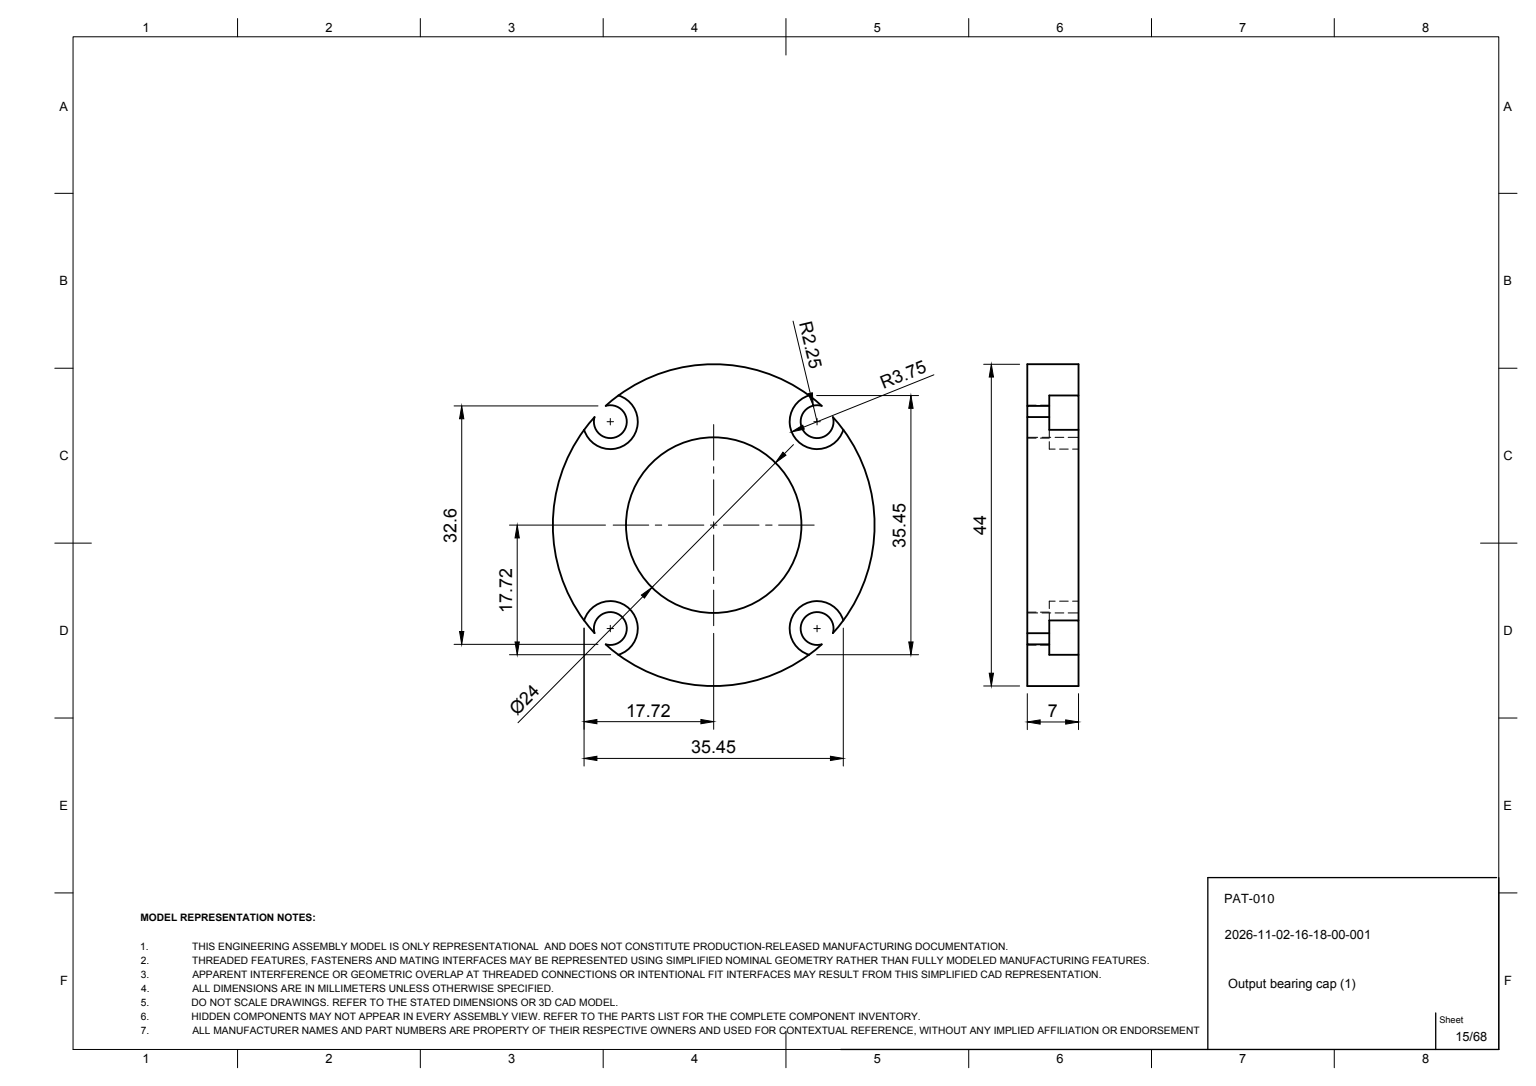
ISO-10303-21;
HEADER;
/* Generated by software containing ST-Developer
 * from STEP Tools, Inc. (www.steptools.com) 
 */

FILE_DESCRIPTION(
/* description */ ('Belt conveyor head drive unit'),
/* implementation_level */ '2;1');

FILE_NAME(
/* name */ 'Output bearing cap (1).step',
/* time_stamp */ '2026-10-28T03:26:19-07:00',
/* author */ (''),
/* organization */ (''),
/* preprocessor_version */ 'ST-DEVELOPER v20.2',
/* originating_system */ 'Autodesk Translation Framework v15.17.0.0',
/* authorisation */ '');

FILE_SCHEMA (('AUTOMOTIVE_DESIGN { 1 0 10303 214 3 1 1 }'));
ENDSEC;

DATA;
#10=MECHANICAL_DESIGN_GEOMETRIC_PRESENTATION_REPRESENTATION('',(#861),#27069);
#723=SHAPE_REPRESENTATION_RELATIONSHIP('SRR','None',#27367,#792);
#792=ADVANCED_BREP_SHAPE_REPRESENTATION('',(#946),#27009);
#861=STYLED_ITEM('',(#27797),#946);
#946=MANIFOLD_SOLID_BREP('Body1',#13726);
#1089=FACE_BOUND('',#2692,.T.);
#1090=FACE_BOUND('',#2694,.T.);
#1361=PLANE('',#14925);
#1362=PLANE('',#14929);
#1363=PLANE('',#14936);
#1364=PLANE('',#14943);
#1365=PLANE('',#14959);
#1366=PLANE('',#14964);
#1802=FACE_OUTER_BOUND('',#2679,.T.);
#1803=FACE_OUTER_BOUND('',#2680,.T.);
#1804=FACE_OUTER_BOUND('',#2681,.T.);
#1805=FACE_OUTER_BOUND('',#2682,.T.);
#1806=FACE_OUTER_BOUND('',#2683,.T.);
#1807=FACE_OUTER_BOUND('',#2684,.T.);
#1808=FACE_OUTER_BOUND('',#2685,.T.);
#1809=FACE_OUTER_BOUND('',#2686,.T.);
#1810=FACE_OUTER_BOUND('',#2687,.T.);
#1811=FACE_OUTER_BOUND('',#2688,.T.);
#1812=FACE_OUTER_BOUND('',#2689,.T.);
#1813=FACE_OUTER_BOUND('',#2690,.T.);
#1814=FACE_OUTER_BOUND('',#2691,.T.);
#1815=FACE_OUTER_BOUND('',#2693,.T.);
#1816=FACE_OUTER_BOUND('',#2695,.T.);
#1817=FACE_OUTER_BOUND('',#2696,.T.);
#1818=FACE_OUTER_BOUND('',#2697,.T.);
#1819=FACE_OUTER_BOUND('',#2698,.T.);
#1820=FACE_OUTER_BOUND('',#2699,.T.);
#2679=EDGE_LOOP('',(#9714,#9715,#9716,#9717));
#2680=EDGE_LOOP('',(#9718,#9719,#9720,#9721));
#2681=EDGE_LOOP('',(#9722,#9723,#9724,#9725));
#2682=EDGE_LOOP('',(#9726,#9727,#9728,#9729));
#2683=EDGE_LOOP('',(#9730,#9731,#9732,#9733));
#2684=EDGE_LOOP('',(#9734,#9735,#9736,#9737));
#2685=EDGE_LOOP('',(#9738,#9739,#9740,#9741));
#2686=EDGE_LOOP('',(#9742,#9743,#9744,#9745));
#2687=EDGE_LOOP('',(#9746,#9747,#9748,#9749));
#2688=EDGE_LOOP('',(#9750,#9751,#9752,#9753));
#2689=EDGE_LOOP('',(#9754,#9755,#9756,#9757));
#2690=EDGE_LOOP('',(#9758,#9759,#9760,#9761,#9762,#9763,#9764,#9765));
#2691=EDGE_LOOP('',(#9766,#9767,#9768,#9769,#9770,#9771,#9772,#9773));
#2692=EDGE_LOOP('',(#9774));
#2693=EDGE_LOOP('',(#9775,#9776,#9777,#9778,#9779,#9780,#9781,#9782));
#2694=EDGE_LOOP('',(#9783));
#2695=EDGE_LOOP('',(#9784,#9785,#9786,#9787,#9788,#9789,#9790,#9791));
#2696=EDGE_LOOP('',(#9792,#9793,#9794,#9795,#9796,#9797,#9798,#9799));
#2697=EDGE_LOOP('',(#9800,#9801,#9802,#9803));
#2698=EDGE_LOOP('',(#9804,#9805,#9806,#9807,#9808,#9809,#9810,#9811));
#2699=EDGE_LOOP('',(#9812,#9813,#9814,#9815));
#3702=LINE('',#21789,#4494);
#3703=LINE('',#21793,#4495);
#3704=LINE('',#21812,#4496);
#3705=LINE('',#21815,#4497);
#3706=LINE('',#21827,#4498);
#3707=LINE('',#21830,#4499);
#3708=LINE('',#21842,#4500);
#3709=LINE('',#21845,#4501);
#3710=LINE('',#21848,#4502);
#3711=LINE('',#21851,#4503);
#3712=LINE('',#21854,#4504);
#3713=LINE('',#21857,#4505);
#3714=LINE('',#21860,#4506);
#3715=LINE('',#21863,#4507);
#3716=LINE('',#21868,#4508);
#3717=LINE('',#21886,#4509);
#3718=LINE('',#21889,#4510);
#4494=VECTOR('',#17360,1.);
#4495=VECTOR('',#17363,1.);
#4496=VECTOR('',#17386,1.);
#4497=VECTOR('',#17389,1.);
#4498=VECTOR('',#17402,1.);
#4499=VECTOR('',#17405,1.);
#4500=VECTOR('',#17418,1.);
#4501=VECTOR('',#17421,1.);
#4502=VECTOR('',#17424,1.);
#4503=VECTOR('',#17427,1.);
#4504=VECTOR('',#17430,1.);
#4505=VECTOR('',#17433,1.);
#4506=VECTOR('',#17436,1.);
#4507=VECTOR('',#17439,1.);
#4508=VECTOR('',#17446,1.);
#4509=VECTOR('',#17475,1.);
#4510=VECTOR('',#17480,1.2);
#5256=CIRCLE('',#14923,0.375);
#5257=CIRCLE('',#14924,0.375);
#5258=CIRCLE('',#14926,2.2);
#5259=CIRCLE('',#14927,0.225);
#5260=CIRCLE('',#14928,2.2);
#5261=CIRCLE('',#14930,2.2);
#5262=CIRCLE('',#14931,0.375);
#5263=CIRCLE('',#14932,2.2);
#5264=CIRCLE('',#14933,0.225);
#5265=CIRCLE('',#14935,0.375);
#5266=CIRCLE('',#14937,2.2);
#5267=CIRCLE('',#14938,0.375);
#5268=CIRCLE('',#14939,2.2);
#5269=CIRCLE('',#14940,0.225);
#5270=CIRCLE('',#14942,0.375);
#5271=CIRCLE('',#14944,2.2);
#5272=CIRCLE('',#14945,0.375);
#5273=CIRCLE('',#14946,2.2);
#5274=CIRCLE('',#14947,0.225);
#5275=CIRCLE('',#14949,0.375);
#5276=CIRCLE('',#14951,0.225);
#5277=CIRCLE('',#14953,0.225);
#5278=CIRCLE('',#14955,0.225);
#5279=CIRCLE('',#14957,2.2);
#5280=CIRCLE('',#14958,2.2);
#5281=CIRCLE('',#14960,2.2);
#5282=CIRCLE('',#14961,2.2);
#5283=CIRCLE('',#14962,2.2);
#5284=CIRCLE('',#14963,1.2);
#5285=CIRCLE('',#14965,0.225);
#5286=CIRCLE('',#14966,2.2);
#5287=CIRCLE('',#14967,2.2);
#5288=CIRCLE('',#14968,2.2);
#5289=CIRCLE('',#14969,1.2);
#6205=VERTEX_POINT('',#21787);
#6206=VERTEX_POINT('',#21788);
#6207=VERTEX_POINT('',#21790);
#6208=VERTEX_POINT('',#21792);
#6209=VERTEX_POINT('',#21796);
#6210=VERTEX_POINT('',#21798);
#6211=VERTEX_POINT('',#21802);
#6212=VERTEX_POINT('',#21803);
#6213=VERTEX_POINT('',#21805);
#6214=VERTEX_POINT('',#21807);
#6215=VERTEX_POINT('',#21811);
#6216=VERTEX_POINT('',#21813);
#6217=VERTEX_POINT('',#21817);
#6218=VERTEX_POINT('',#21818);
#6219=VERTEX_POINT('',#21820);
#6220=VERTEX_POINT('',#21822);
#6221=VERTEX_POINT('',#21826);
#6222=VERTEX_POINT('',#21828);
#6223=VERTEX_POINT('',#21832);
#6224=VERTEX_POINT('',#21833);
#6225=VERTEX_POINT('',#21835);
#6226=VERTEX_POINT('',#21837);
#6227=VERTEX_POINT('',#21841);
#6228=VERTEX_POINT('',#21843);
#6229=VERTEX_POINT('',#21847);
#6230=VERTEX_POINT('',#21849);
#6231=VERTEX_POINT('',#21853);
#6232=VERTEX_POINT('',#21855);
#6233=VERTEX_POINT('',#21859);
#6234=VERTEX_POINT('',#21861);
#6235=VERTEX_POINT('',#21866);
#6236=VERTEX_POINT('',#21873);
#6237=VERTEX_POINT('',#21876);
#6238=VERTEX_POINT('',#21881);
#7549=EDGE_CURVE('',#6205,#6206,#3702,.T.);
#7550=EDGE_CURVE('',#6207,#6205,#5256,.T.);
#7551=EDGE_CURVE('',#6208,#6207,#3703,.T.);
#7552=EDGE_CURVE('',#6206,#6208,#5257,.T.);
#7553=EDGE_CURVE('',#6209,#6205,#5258,.T.);
#7554=EDGE_CURVE('',#6210,#6209,#5259,.T.);
#7555=EDGE_CURVE('',#6207,#6210,#5260,.T.);
#7556=EDGE_CURVE('',#6211,#6212,#5261,.T.);
#7557=EDGE_CURVE('',#6211,#6213,#5262,.T.);
#7558=EDGE_CURVE('',#6214,#6213,#5263,.T.);
#7559=EDGE_CURVE('',#6212,#6214,#5264,.T.);
#7560=EDGE_CURVE('',#6215,#6211,#3704,.T.);
#7561=EDGE_CURVE('',#6216,#6215,#5265,.T.);
#7562=EDGE_CURVE('',#6213,#6216,#3705,.T.);
#7563=EDGE_CURVE('',#6217,#6218,#5266,.T.);
#7564=EDGE_CURVE('',#6217,#6219,#5267,.T.);
#7565=EDGE_CURVE('',#6220,#6219,#5268,.T.);
#7566=EDGE_CURVE('',#6218,#6220,#5269,.T.);
#7567=EDGE_CURVE('',#6221,#6217,#3706,.T.);
#7568=EDGE_CURVE('',#6222,#6221,#5270,.T.);
#7569=EDGE_CURVE('',#6219,#6222,#3707,.T.);
#7570=EDGE_CURVE('',#6223,#6224,#5271,.T.);
#7571=EDGE_CURVE('',#6223,#6225,#5272,.T.);
#7572=EDGE_CURVE('',#6226,#6225,#5273,.T.);
#7573=EDGE_CURVE('',#6224,#6226,#5274,.T.);
#7574=EDGE_CURVE('',#6227,#6223,#3708,.T.);
#7575=EDGE_CURVE('',#6228,#6227,#5275,.T.);
#7576=EDGE_CURVE('',#6225,#6228,#3709,.T.);
#7577=EDGE_CURVE('',#6229,#6214,#3710,.T.);
#7578=EDGE_CURVE('',#6230,#6229,#5276,.T.);
#7579=EDGE_CURVE('',#6212,#6230,#3711,.T.);
#7580=EDGE_CURVE('',#6231,#6220,#3712,.T.);
#7581=EDGE_CURVE('',#6232,#6231,#5277,.T.);
#7582=EDGE_CURVE('',#6218,#6232,#3713,.T.);
#7583=EDGE_CURVE('',#6233,#6226,#3714,.T.);
#7584=EDGE_CURVE('',#6234,#6233,#5278,.T.);
#7585=EDGE_CURVE('',#6224,#6234,#3715,.T.);
#7586=EDGE_CURVE('',#6227,#6206,#5279,.T.);
#7587=EDGE_CURVE('',#6234,#6235,#5280,.T.);
#7588=EDGE_CURVE('',#6235,#6209,#3716,.T.);
#7589=EDGE_CURVE('',#6208,#6216,#5281,.T.);
#7590=EDGE_CURVE('',#6215,#6222,#5282,.T.);
#7591=EDGE_CURVE('',#6221,#6228,#5283,.T.);
#7592=EDGE_CURVE('',#6236,#6236,#5284,.T.);
#7593=EDGE_CURVE('',#6237,#6235,#5285,.T.);
#7594=EDGE_CURVE('',#6232,#6233,#5286,.T.);
#7595=EDGE_CURVE('',#6230,#6231,#5287,.T.);
#7596=EDGE_CURVE('',#6237,#6229,#5288,.T.);
#7597=EDGE_CURVE('',#6238,#6238,#5289,.T.);
#7598=EDGE_CURVE('',#6210,#6237,#3717,.T.);
#7599=EDGE_CURVE('',#6236,#6238,#3718,.T.);
#9714=ORIENTED_EDGE('',*,*,#7549,.F.);
#9715=ORIENTED_EDGE('',*,*,#7550,.F.);
#9716=ORIENTED_EDGE('',*,*,#7551,.F.);
#9717=ORIENTED_EDGE('',*,*,#7552,.F.);
#9718=ORIENTED_EDGE('',*,*,#7553,.F.);
#9719=ORIENTED_EDGE('',*,*,#7554,.F.);
#9720=ORIENTED_EDGE('',*,*,#7555,.F.);
#9721=ORIENTED_EDGE('',*,*,#7550,.T.);
#9722=ORIENTED_EDGE('',*,*,#7556,.F.);
#9723=ORIENTED_EDGE('',*,*,#7557,.T.);
#9724=ORIENTED_EDGE('',*,*,#7558,.F.);
#9725=ORIENTED_EDGE('',*,*,#7559,.F.);
#9726=ORIENTED_EDGE('',*,*,#7560,.F.);
#9727=ORIENTED_EDGE('',*,*,#7561,.F.);
#9728=ORIENTED_EDGE('',*,*,#7562,.F.);
#9729=ORIENTED_EDGE('',*,*,#7557,.F.);
#9730=ORIENTED_EDGE('',*,*,#7563,.F.);
#9731=ORIENTED_EDGE('',*,*,#7564,.T.);
#9732=ORIENTED_EDGE('',*,*,#7565,.F.);
#9733=ORIENTED_EDGE('',*,*,#7566,.F.);
#9734=ORIENTED_EDGE('',*,*,#7567,.F.);
#9735=ORIENTED_EDGE('',*,*,#7568,.F.);
#9736=ORIENTED_EDGE('',*,*,#7569,.F.);
#9737=ORIENTED_EDGE('',*,*,#7564,.F.);
#9738=ORIENTED_EDGE('',*,*,#7570,.F.);
#9739=ORIENTED_EDGE('',*,*,#7571,.T.);
#9740=ORIENTED_EDGE('',*,*,#7572,.F.);
#9741=ORIENTED_EDGE('',*,*,#7573,.F.);
#9742=ORIENTED_EDGE('',*,*,#7574,.F.);
#9743=ORIENTED_EDGE('',*,*,#7575,.F.);
#9744=ORIENTED_EDGE('',*,*,#7576,.F.);
#9745=ORIENTED_EDGE('',*,*,#7571,.F.);
#9746=ORIENTED_EDGE('',*,*,#7559,.T.);
#9747=ORIENTED_EDGE('',*,*,#7577,.F.);
#9748=ORIENTED_EDGE('',*,*,#7578,.F.);
#9749=ORIENTED_EDGE('',*,*,#7579,.F.);
#9750=ORIENTED_EDGE('',*,*,#7566,.T.);
#9751=ORIENTED_EDGE('',*,*,#7580,.F.);
#9752=ORIENTED_EDGE('',*,*,#7581,.F.);
#9753=ORIENTED_EDGE('',*,*,#7582,.F.);
#9754=ORIENTED_EDGE('',*,*,#7573,.T.);
#9755=ORIENTED_EDGE('',*,*,#7583,.F.);
#9756=ORIENTED_EDGE('',*,*,#7584,.F.);
#9757=ORIENTED_EDGE('',*,*,#7585,.F.);
#9758=ORIENTED_EDGE('',*,*,#7553,.T.);
#9759=ORIENTED_EDGE('',*,*,#7549,.T.);
#9760=ORIENTED_EDGE('',*,*,#7586,.F.);
#9761=ORIENTED_EDGE('',*,*,#7574,.T.);
#9762=ORIENTED_EDGE('',*,*,#7570,.T.);
#9763=ORIENTED_EDGE('',*,*,#7585,.T.);
#9764=ORIENTED_EDGE('',*,*,#7587,.T.);
#9765=ORIENTED_EDGE('',*,*,#7588,.T.);
#9766=ORIENTED_EDGE('',*,*,#7552,.T.);
#9767=ORIENTED_EDGE('',*,*,#7589,.T.);
#9768=ORIENTED_EDGE('',*,*,#7561,.T.);
#9769=ORIENTED_EDGE('',*,*,#7590,.T.);
#9770=ORIENTED_EDGE('',*,*,#7568,.T.);
#9771=ORIENTED_EDGE('',*,*,#7591,.T.);
#9772=ORIENTED_EDGE('',*,*,#7575,.T.);
#9773=ORIENTED_EDGE('',*,*,#7586,.T.);
#9774=ORIENTED_EDGE('',*,*,#7592,.T.);
#9775=ORIENTED_EDGE('',*,*,#7593,.T.);
#9776=ORIENTED_EDGE('',*,*,#7587,.F.);
#9777=ORIENTED_EDGE('',*,*,#7584,.T.);
#9778=ORIENTED_EDGE('',*,*,#7594,.F.);
#9779=ORIENTED_EDGE('',*,*,#7581,.T.);
#9780=ORIENTED_EDGE('',*,*,#7595,.F.);
#9781=ORIENTED_EDGE('',*,*,#7578,.T.);
#9782=ORIENTED_EDGE('',*,*,#7596,.F.);
#9783=ORIENTED_EDGE('',*,*,#7597,.F.);
#9784=ORIENTED_EDGE('',*,*,#7563,.T.);
#9785=ORIENTED_EDGE('',*,*,#7582,.T.);
#9786=ORIENTED_EDGE('',*,*,#7594,.T.);
#9787=ORIENTED_EDGE('',*,*,#7583,.T.);
#9788=ORIENTED_EDGE('',*,*,#7572,.T.);
#9789=ORIENTED_EDGE('',*,*,#7576,.T.);
#9790=ORIENTED_EDGE('',*,*,#7591,.F.);
#9791=ORIENTED_EDGE('',*,*,#7567,.T.);
#9792=ORIENTED_EDGE('',*,*,#7556,.T.);
#9793=ORIENTED_EDGE('',*,*,#7579,.T.);
#9794=ORIENTED_EDGE('',*,*,#7595,.T.);
#9795=ORIENTED_EDGE('',*,*,#7580,.T.);
#9796=ORIENTED_EDGE('',*,*,#7565,.T.);
#9797=ORIENTED_EDGE('',*,*,#7569,.T.);
#9798=ORIENTED_EDGE('',*,*,#7590,.F.);
#9799=ORIENTED_EDGE('',*,*,#7560,.T.);
#9800=ORIENTED_EDGE('',*,*,#7554,.T.);
#9801=ORIENTED_EDGE('',*,*,#7588,.F.);
#9802=ORIENTED_EDGE('',*,*,#7593,.F.);
#9803=ORIENTED_EDGE('',*,*,#7598,.F.);
#9804=ORIENTED_EDGE('',*,*,#7555,.T.);
#9805=ORIENTED_EDGE('',*,*,#7598,.T.);
#9806=ORIENTED_EDGE('',*,*,#7596,.T.);
#9807=ORIENTED_EDGE('',*,*,#7577,.T.);
#9808=ORIENTED_EDGE('',*,*,#7558,.T.);
#9809=ORIENTED_EDGE('',*,*,#7562,.T.);
#9810=ORIENTED_EDGE('',*,*,#7589,.F.);
#9811=ORIENTED_EDGE('',*,*,#7551,.T.);
#9812=ORIENTED_EDGE('',*,*,#7592,.F.);
#9813=ORIENTED_EDGE('',*,*,#7599,.T.);
#9814=ORIENTED_EDGE('',*,*,#7597,.T.);
#9815=ORIENTED_EDGE('',*,*,#7599,.F.);
#12617=CYLINDRICAL_SURFACE('',#14922,0.375);
#12618=CYLINDRICAL_SURFACE('',#14934,0.375);
#12619=CYLINDRICAL_SURFACE('',#14941,0.375);
#12620=CYLINDRICAL_SURFACE('',#14948,0.375);
#12621=CYLINDRICAL_SURFACE('',#14950,0.225);
#12622=CYLINDRICAL_SURFACE('',#14952,0.225);
#12623=CYLINDRICAL_SURFACE('',#14954,0.225);
#12624=CYLINDRICAL_SURFACE('',#14956,2.2);
#12625=CYLINDRICAL_SURFACE('',#14970,2.2);
#12626=CYLINDRICAL_SURFACE('',#14971,2.2);
#12627=CYLINDRICAL_SURFACE('',#14972,0.225);
#12628=CYLINDRICAL_SURFACE('',#14973,2.2);
#12629=CYLINDRICAL_SURFACE('',#14974,1.2);
#13081=ADVANCED_FACE('',(#1802),#12617,.F.);
#13082=ADVANCED_FACE('',(#1803),#1361,.T.);
#13083=ADVANCED_FACE('',(#1804),#1362,.T.);
#13084=ADVANCED_FACE('',(#1805),#12618,.F.);
#13085=ADVANCED_FACE('',(#1806),#1363,.T.);
#13086=ADVANCED_FACE('',(#1807),#12619,.F.);
#13087=ADVANCED_FACE('',(#1808),#1364,.T.);
#13088=ADVANCED_FACE('',(#1809),#12620,.F.);
#13089=ADVANCED_FACE('',(#1810),#12621,.F.);
#13090=ADVANCED_FACE('',(#1811),#12622,.F.);
#13091=ADVANCED_FACE('',(#1812),#12623,.F.);
#13092=ADVANCED_FACE('',(#1813),#12624,.T.);
#13093=ADVANCED_FACE('',(#1814,#1089),#1365,.T.);
#13094=ADVANCED_FACE('',(#1815,#1090),#1366,.F.);
#13095=ADVANCED_FACE('',(#1816),#12625,.T.);
#13096=ADVANCED_FACE('',(#1817),#12626,.T.);
#13097=ADVANCED_FACE('',(#1818),#12627,.F.);
#13098=ADVANCED_FACE('',(#1819),#12628,.T.);
#13099=ADVANCED_FACE('',(#1820),#12629,.F.);
#13726=CLOSED_SHELL('',(#13081,#13082,#13083,#13084,#13085,#13086,#13087,
#13088,#13089,#13090,#13091,#13092,#13093,#13094,#13095,#13096,#13097,#13098,
#13099));
#14921=AXIS2_PLACEMENT_3D('',#21785,#17356,#17357);
#14922=AXIS2_PLACEMENT_3D('',#21786,#17358,#17359);
#14923=AXIS2_PLACEMENT_3D('',#21791,#17361,#17362);
#14924=AXIS2_PLACEMENT_3D('',#21794,#17364,#17365);
#14925=AXIS2_PLACEMENT_3D('',#21795,#17366,#17367);
#14926=AXIS2_PLACEMENT_3D('',#21797,#17368,#17369);
#14927=AXIS2_PLACEMENT_3D('',#21799,#17370,#17371);
#14928=AXIS2_PLACEMENT_3D('',#21800,#17372,#17373);
#14929=AXIS2_PLACEMENT_3D('',#21801,#17374,#17375);
#14930=AXIS2_PLACEMENT_3D('',#21804,#17376,#17377);
#14931=AXIS2_PLACEMENT_3D('',#21806,#17378,#17379);
#14932=AXIS2_PLACEMENT_3D('',#21808,#17380,#17381);
#14933=AXIS2_PLACEMENT_3D('',#21809,#17382,#17383);
#14934=AXIS2_PLACEMENT_3D('',#21810,#17384,#17385);
#14935=AXIS2_PLACEMENT_3D('',#21814,#17387,#17388);
#14936=AXIS2_PLACEMENT_3D('',#21816,#17390,#17391);
#14937=AXIS2_PLACEMENT_3D('',#21819,#17392,#17393);
#14938=AXIS2_PLACEMENT_3D('',#21821,#17394,#17395);
#14939=AXIS2_PLACEMENT_3D('',#21823,#17396,#17397);
#14940=AXIS2_PLACEMENT_3D('',#21824,#17398,#17399);
#14941=AXIS2_PLACEMENT_3D('',#21825,#17400,#17401);
#14942=AXIS2_PLACEMENT_3D('',#21829,#17403,#17404);
#14943=AXIS2_PLACEMENT_3D('',#21831,#17406,#17407);
#14944=AXIS2_PLACEMENT_3D('',#21834,#17408,#17409);
#14945=AXIS2_PLACEMENT_3D('',#21836,#17410,#17411);
#14946=AXIS2_PLACEMENT_3D('',#21838,#17412,#17413);
#14947=AXIS2_PLACEMENT_3D('',#21839,#17414,#17415);
#14948=AXIS2_PLACEMENT_3D('',#21840,#17416,#17417);
#14949=AXIS2_PLACEMENT_3D('',#21844,#17419,#17420);
#14950=AXIS2_PLACEMENT_3D('',#21846,#17422,#17423);
#14951=AXIS2_PLACEMENT_3D('',#21850,#17425,#17426);
#14952=AXIS2_PLACEMENT_3D('',#21852,#17428,#17429);
#14953=AXIS2_PLACEMENT_3D('',#21856,#17431,#17432);
#14954=AXIS2_PLACEMENT_3D('',#21858,#17434,#17435);
#14955=AXIS2_PLACEMENT_3D('',#21862,#17437,#17438);
#14956=AXIS2_PLACEMENT_3D('',#21864,#17440,#17441);
#14957=AXIS2_PLACEMENT_3D('',#21865,#17442,#17443);
#14958=AXIS2_PLACEMENT_3D('',#21867,#17444,#17445);
#14959=AXIS2_PLACEMENT_3D('',#21869,#17447,#17448);
#14960=AXIS2_PLACEMENT_3D('',#21870,#17449,#17450);
#14961=AXIS2_PLACEMENT_3D('',#21871,#17451,#17452);
#14962=AXIS2_PLACEMENT_3D('',#21872,#17453,#17454);
#14963=AXIS2_PLACEMENT_3D('',#21874,#17455,#17456);
#14964=AXIS2_PLACEMENT_3D('',#21875,#17457,#17458);
#14965=AXIS2_PLACEMENT_3D('',#21877,#17459,#17460);
#14966=AXIS2_PLACEMENT_3D('',#21878,#17461,#17462);
#14967=AXIS2_PLACEMENT_3D('',#21879,#17463,#17464);
#14968=AXIS2_PLACEMENT_3D('',#21880,#17465,#17466);
#14969=AXIS2_PLACEMENT_3D('',#21882,#17467,#17468);
#14970=AXIS2_PLACEMENT_3D('',#21883,#17469,#17470);
#14971=AXIS2_PLACEMENT_3D('',#21884,#17471,#17472);
#14972=AXIS2_PLACEMENT_3D('',#21885,#17473,#17474);
#14973=AXIS2_PLACEMENT_3D('',#21887,#17476,#17477);
#14974=AXIS2_PLACEMENT_3D('',#21888,#17478,#17479);
#17356=DIRECTION('axis',(0.,0.,1.));
#17357=DIRECTION('refdir',(1.,0.,0.));
#17358=DIRECTION('center_axis',(0.,1.,0.));
#17359=DIRECTION('ref_axis',(1.,0.,0.));
#17360=DIRECTION('',(0.,1.,0.));
#17361=DIRECTION('center_axis',(0.,1.,0.));
#17362=DIRECTION('ref_axis',(1.,0.,0.));
#17363=DIRECTION('',(0.,-1.,0.));
#17364=DIRECTION('center_axis',(0.,-1.,0.));
#17365=DIRECTION('ref_axis',(1.,0.,0.));
#17366=DIRECTION('center_axis',(0.,1.,0.));
#17367=DIRECTION('ref_axis',(1.,0.,0.));
#17368=DIRECTION('center_axis',(0.,-1.,0.));
#17369=DIRECTION('ref_axis',(1.,0.,0.));
#17370=DIRECTION('center_axis',(0.,1.,0.));
#17371=DIRECTION('ref_axis',(1.,0.,0.));
#17372=DIRECTION('center_axis',(0.,-1.,0.));
#17373=DIRECTION('ref_axis',(1.,0.,0.));
#17374=DIRECTION('center_axis',(0.,1.,0.));
#17375=DIRECTION('ref_axis',(1.,0.,0.));
#17376=DIRECTION('center_axis',(0.,-1.,0.));
#17377=DIRECTION('ref_axis',(1.,0.,0.));
#17378=DIRECTION('center_axis',(0.,1.,0.));
#17379=DIRECTION('ref_axis',(1.,0.,0.));
#17380=DIRECTION('center_axis',(0.,-1.,0.));
#17381=DIRECTION('ref_axis',(1.,0.,0.));
#17382=DIRECTION('center_axis',(0.,1.,0.));
#17383=DIRECTION('ref_axis',(1.,0.,0.));
#17384=DIRECTION('center_axis',(0.,1.,0.));
#17385=DIRECTION('ref_axis',(1.,0.,0.));
#17386=DIRECTION('',(0.,-1.,0.));
#17387=DIRECTION('center_axis',(0.,-1.,0.));
#17388=DIRECTION('ref_axis',(1.,0.,0.));
#17389=DIRECTION('',(0.,1.,0.));
#17390=DIRECTION('center_axis',(0.,1.,0.));
#17391=DIRECTION('ref_axis',(1.,0.,0.));
#17392=DIRECTION('center_axis',(0.,-1.,0.));
#17393=DIRECTION('ref_axis',(1.,0.,0.));
#17394=DIRECTION('center_axis',(0.,1.,0.));
#17395=DIRECTION('ref_axis',(1.,0.,0.));
#17396=DIRECTION('center_axis',(0.,-1.,0.));
#17397=DIRECTION('ref_axis',(1.,0.,0.));
#17398=DIRECTION('center_axis',(0.,1.,0.));
#17399=DIRECTION('ref_axis',(1.,0.,0.));
#17400=DIRECTION('center_axis',(0.,1.,0.));
#17401=DIRECTION('ref_axis',(-0.707106781186547,0.,-0.707106781186548));
#17402=DIRECTION('',(0.,-1.,0.));
#17403=DIRECTION('center_axis',(0.,-1.,0.));
#17404=DIRECTION('ref_axis',(1.,0.,0.));
#17405=DIRECTION('',(0.,1.,0.));
#17406=DIRECTION('center_axis',(0.,1.,0.));
#17407=DIRECTION('ref_axis',(1.,0.,0.));
#17408=DIRECTION('center_axis',(0.,-1.,0.));
#17409=DIRECTION('ref_axis',(1.,0.,0.));
#17410=DIRECTION('center_axis',(0.,1.,0.));
#17411=DIRECTION('ref_axis',(1.,0.,0.));
#17412=DIRECTION('center_axis',(0.,-1.,0.));
#17413=DIRECTION('ref_axis',(1.,0.,0.));
#17414=DIRECTION('center_axis',(0.,1.,0.));
#17415=DIRECTION('ref_axis',(1.,0.,0.));
#17416=DIRECTION('center_axis',(0.,1.,0.));
#17417=DIRECTION('ref_axis',(-0.707106781186548,0.,0.707106781186547));
#17418=DIRECTION('',(0.,-1.,0.));
#17419=DIRECTION('center_axis',(0.,-1.,0.));
#17420=DIRECTION('ref_axis',(1.,0.,0.));
#17421=DIRECTION('',(0.,1.,0.));
#17422=DIRECTION('center_axis',(0.,1.,0.));
#17423=DIRECTION('ref_axis',(0.707106781186545,0.,-0.70710678118655));
#17424=DIRECTION('',(0.,1.,0.));
#17425=DIRECTION('center_axis',(0.,1.,0.));
#17426=DIRECTION('ref_axis',(1.,0.,0.));
#17427=DIRECTION('',(0.,-1.,0.));
#17428=DIRECTION('center_axis',(0.,1.,0.));
#17429=DIRECTION('ref_axis',(-0.707106781186547,0.,-0.707106781186548));
#17430=DIRECTION('',(0.,1.,0.));
#17431=DIRECTION('center_axis',(0.,1.,0.));
#17432=DIRECTION('ref_axis',(1.,0.,0.));
#17433=DIRECTION('',(0.,-1.,0.));
#17434=DIRECTION('center_axis',(0.,1.,0.));
#17435=DIRECTION('ref_axis',(-0.707106781186544,0.,0.707106781186551));
#17436=DIRECTION('',(0.,1.,0.));
#17437=DIRECTION('center_axis',(0.,1.,0.));
#17438=DIRECTION('ref_axis',(1.,0.,0.));
#17439=DIRECTION('',(0.,-1.,0.));
#17440=DIRECTION('center_axis',(0.,1.,0.));
#17441=DIRECTION('ref_axis',(1.,0.,0.));
#17442=DIRECTION('center_axis',(0.,1.,0.));
#17443=DIRECTION('ref_axis',(1.,0.,0.));
#17444=DIRECTION('center_axis',(0.,1.,0.));
#17445=DIRECTION('ref_axis',(1.,0.,0.));
#17446=DIRECTION('',(0.,1.,0.));
#17447=DIRECTION('center_axis',(0.,1.,0.));
#17448=DIRECTION('ref_axis',(1.,0.,0.));
#17449=DIRECTION('center_axis',(0.,1.,0.));
#17450=DIRECTION('ref_axis',(1.,0.,0.));
#17451=DIRECTION('center_axis',(0.,1.,0.));
#17452=DIRECTION('ref_axis',(1.,0.,0.));
#17453=DIRECTION('center_axis',(0.,1.,0.));
#17454=DIRECTION('ref_axis',(1.,0.,0.));
#17455=DIRECTION('center_axis',(0.,-1.,0.));
#17456=DIRECTION('ref_axis',(1.,0.,0.));
#17457=DIRECTION('center_axis',(0.,1.,0.));
#17458=DIRECTION('ref_axis',(1.,0.,0.));
#17459=DIRECTION('center_axis',(0.,1.,0.));
#17460=DIRECTION('ref_axis',(1.,0.,0.));
#17461=DIRECTION('center_axis',(0.,1.,0.));
#17462=DIRECTION('ref_axis',(1.,0.,0.));
#17463=DIRECTION('center_axis',(0.,1.,0.));
#17464=DIRECTION('ref_axis',(1.,0.,0.));
#17465=DIRECTION('center_axis',(0.,1.,0.));
#17466=DIRECTION('ref_axis',(1.,0.,0.));
#17467=DIRECTION('center_axis',(0.,-1.,0.));
#17468=DIRECTION('ref_axis',(1.,0.,0.));
#17469=DIRECTION('center_axis',(0.,1.,0.));
#17470=DIRECTION('ref_axis',(1.,0.,0.));
#17471=DIRECTION('center_axis',(0.,1.,0.));
#17472=DIRECTION('ref_axis',(1.,0.,0.));
#17473=DIRECTION('center_axis',(0.,1.,0.));
#17474=DIRECTION('ref_axis',(0.707106781186544,0.,0.707106781186551));
#17475=DIRECTION('',(0.,-1.,0.));
#17476=DIRECTION('center_axis',(0.,1.,0.));
#17477=DIRECTION('ref_axis',(-1.,0.,-1.01064309961486E-15));
#17478=DIRECTION('center_axis',(0.,1.,0.));
#17479=DIRECTION('ref_axis',(1.,0.,0.));
#17480=DIRECTION('',(0.,-1.,0.));
#21785=CARTESIAN_POINT('',(0.,0.,0.));
#21786=CARTESIAN_POINT('Origin',(5.55669646780806,1.7,5.58578643762691));
#21787=CARTESIAN_POINT('',(5.66764231833408,1.7,5.22757418455471));
#21788=CARTESIAN_POINT('',(5.66764231833408,2.1,5.22757418455471));
#21789=CARTESIAN_POINT('',(5.66764231833408,1.7,5.22757418455471));
#21790=CARTESIAN_POINT('',(5.19848421473587,1.7,5.69673228815293));
#21791=CARTESIAN_POINT('Origin',(5.55669646780806,1.7,5.58578643762691));
#21792=CARTESIAN_POINT('',(5.19848421473587,2.1,5.69673228815293));
#21793=CARTESIAN_POINT('',(5.19848421473587,1.7,5.69673228815293));
#21794=CARTESIAN_POINT('Origin',(5.55669646780806,2.1,5.58578643762691));
#21795=CARTESIAN_POINT('Origin',(5.55669646780806,1.7,5.58578643762691));
#21796=CARTESIAN_POINT('',(5.49357471024299,1.7,5.36982198749241));
#21797=CARTESIAN_POINT('Origin',(6.97091003018116,1.7,7.));
#21798=CARTESIAN_POINT('',(5.34073201767356,1.7,5.52266468006184));
#21799=CARTESIAN_POINT('Origin',(5.55669646780806,1.7,5.58578643762691));
#21800=CARTESIAN_POINT('Origin',(6.97091003018116,1.7,7.));
#21801=CARTESIAN_POINT('Origin',(5.55669646780806,1.7,8.4142135623731));
#21802=CARTESIAN_POINT('',(5.66764231833408,1.7,8.77242581544529));
#21803=CARTESIAN_POINT('',(5.493574710243,1.7,8.6301780125076));
#21804=CARTESIAN_POINT('Origin',(6.97091003018116,1.7,7.));
#21805=CARTESIAN_POINT('',(5.19848421473587,1.7,8.30326771184707));
#21806=CARTESIAN_POINT('Origin',(5.55669646780806,1.7,8.4142135623731));
#21807=CARTESIAN_POINT('',(5.34073201767356,1.7,8.47733531993816));
#21808=CARTESIAN_POINT('Origin',(6.97091003018116,1.7,7.));
#21809=CARTESIAN_POINT('Origin',(5.55669646780806,1.7,8.4142135623731));
#21810=CARTESIAN_POINT('Origin',(5.55669646780806,1.7,8.4142135623731));
#21811=CARTESIAN_POINT('',(5.66764231833409,2.1,8.77242581544529));
#21812=CARTESIAN_POINT('',(5.66764231833408,1.7,8.77242581544529));
#21813=CARTESIAN_POINT('',(5.19848421473587,2.1,8.30326771184707));
#21814=CARTESIAN_POINT('Origin',(5.55669646780806,2.1,8.4142135623731));
#21815=CARTESIAN_POINT('',(5.19848421473587,1.7,8.30326771184707));
#21816=CARTESIAN_POINT('Origin',(8.38512359255425,1.7,8.4142135623731));
#21817=CARTESIAN_POINT('',(8.74333584562645,1.7,8.30326771184707));
#21818=CARTESIAN_POINT('',(8.60108804268875,1.7,8.47733531993816));
#21819=CARTESIAN_POINT('Origin',(6.97091003018116,1.7,7.));
#21820=CARTESIAN_POINT('',(8.27417774202823,1.7,8.77242581544529));
#21821=CARTESIAN_POINT('Origin',(8.38512359255425,1.7,8.4142135623731));
#21822=CARTESIAN_POINT('',(8.44824535011932,1.7,8.6301780125076));
#21823=CARTESIAN_POINT('Origin',(6.97091003018116,1.7,7.));
#21824=CARTESIAN_POINT('Origin',(8.38512359255425,1.7,8.4142135623731));
#21825=CARTESIAN_POINT('Origin',(8.38512359255425,1.7,8.4142135623731));
#21826=CARTESIAN_POINT('',(8.74333584562645,2.1,8.30326771184707));
#21827=CARTESIAN_POINT('',(8.74333584562645,1.7,8.30326771184707));
#21828=CARTESIAN_POINT('',(8.27417774202823,2.1,8.77242581544529));
#21829=CARTESIAN_POINT('Origin',(8.38512359255425,2.1,8.4142135623731));
#21830=CARTESIAN_POINT('',(8.27417774202823,1.7,8.77242581544529));
#21831=CARTESIAN_POINT('Origin',(8.38512359255425,1.7,5.58578643762691));
#21832=CARTESIAN_POINT('',(8.27417774202823,1.7,5.22757418455471));
#21833=CARTESIAN_POINT('',(8.44824535011932,1.7,5.36982198749241));
#21834=CARTESIAN_POINT('Origin',(6.97091003018116,1.7,7.));
#21835=CARTESIAN_POINT('',(8.74333584562644,1.7,5.69673228815293));
#21836=CARTESIAN_POINT('Origin',(8.38512359255425,1.7,5.58578643762691));
#21837=CARTESIAN_POINT('',(8.60108804268875,1.7,5.52266468006184));
#21838=CARTESIAN_POINT('Origin',(6.97091003018116,1.7,7.));
#21839=CARTESIAN_POINT('Origin',(8.38512359255425,1.7,5.58578643762691));
#21840=CARTESIAN_POINT('Origin',(8.38512359255425,1.7,5.58578643762691));
#21841=CARTESIAN_POINT('',(8.27417774202823,2.1,5.22757418455471));
#21842=CARTESIAN_POINT('',(8.27417774202823,1.7,5.22757418455471));
#21843=CARTESIAN_POINT('',(8.74333584562644,2.1,5.69673228815293));
#21844=CARTESIAN_POINT('Origin',(8.38512359255425,2.1,5.58578643762691));
#21845=CARTESIAN_POINT('',(8.74333584562644,1.7,5.69673228815293));
#21846=CARTESIAN_POINT('Origin',(5.55669646780806,1.7,8.4142135623731));
#21847=CARTESIAN_POINT('',(5.34073201767356,1.4,8.47733531993816));
#21848=CARTESIAN_POINT('',(5.34073201767356,1.7,8.47733531993816));
#21849=CARTESIAN_POINT('',(5.493574710243,1.4,8.6301780125076));
#21850=CARTESIAN_POINT('Origin',(5.55669646780806,1.4,8.4142135623731));
#21851=CARTESIAN_POINT('',(5.493574710243,1.3,8.6301780125076));
#21852=CARTESIAN_POINT('Origin',(8.38512359255425,1.7,8.4142135623731));
#21853=CARTESIAN_POINT('',(8.44824535011931,1.4,8.6301780125076));
#21854=CARTESIAN_POINT('',(8.44824535011932,1.7,8.6301780125076));
#21855=CARTESIAN_POINT('',(8.60108804268875,1.4,8.47733531993816));
#21856=CARTESIAN_POINT('Origin',(8.38512359255425,1.4,8.4142135623731));
#21857=CARTESIAN_POINT('',(8.60108804268875,1.3,8.47733531993816));
#21858=CARTESIAN_POINT('Origin',(8.38512359255425,1.7,5.58578643762691));
#21859=CARTESIAN_POINT('',(8.60108804268875,1.4,5.52266468006184));
#21860=CARTESIAN_POINT('',(8.60108804268875,1.7,5.52266468006184));
#21861=CARTESIAN_POINT('',(8.44824535011932,1.4,5.36982198749241));
#21862=CARTESIAN_POINT('Origin',(8.38512359255425,1.4,5.58578643762691));
#21863=CARTESIAN_POINT('',(8.44824535011932,1.3,5.36982198749241));
#21864=CARTESIAN_POINT('Origin',(6.97091003018116,1.8,7.));
#21865=CARTESIAN_POINT('Origin',(6.97091003018116,2.1,7.));
#21866=CARTESIAN_POINT('',(5.49357471024299,1.4,5.36982198749241));
#21867=CARTESIAN_POINT('Origin',(6.97091003018116,1.4,7.));
#21868=CARTESIAN_POINT('',(5.49357471024299,1.7,5.36982198749241));
#21869=CARTESIAN_POINT('Origin',(6.97091003018116,2.1,7.));
#21870=CARTESIAN_POINT('Origin',(6.97091003018116,2.1,7.));
#21871=CARTESIAN_POINT('Origin',(6.97091003018116,2.1,7.));
#21872=CARTESIAN_POINT('Origin',(6.97091003018116,2.1,7.));
#21873=CARTESIAN_POINT('',(5.77091003018116,2.1,7.));
#21874=CARTESIAN_POINT('Origin',(6.97091003018116,2.1,7.));
#21875=CARTESIAN_POINT('Origin',(6.97091003018116,1.4,7.));
#21876=CARTESIAN_POINT('',(5.34073201767356,1.4,5.52266468006184));
#21877=CARTESIAN_POINT('Origin',(5.55669646780806,1.4,5.58578643762691));
#21878=CARTESIAN_POINT('Origin',(6.97091003018116,1.4,7.));
#21879=CARTESIAN_POINT('Origin',(6.97091003018116,1.4,7.));
#21880=CARTESIAN_POINT('Origin',(6.97091003018116,1.4,7.));
#21881=CARTESIAN_POINT('',(5.77091003018116,1.4,7.));
#21882=CARTESIAN_POINT('Origin',(6.97091003018116,1.4,7.));
#21883=CARTESIAN_POINT('Origin',(6.97091003018116,1.8,7.));
#21884=CARTESIAN_POINT('Origin',(6.97091003018116,1.8,7.));
#21885=CARTESIAN_POINT('Origin',(5.55669646780806,1.7,5.58578643762691));
#21886=CARTESIAN_POINT('',(5.34073201767356,1.3,5.52266468006184));
#21887=CARTESIAN_POINT('Origin',(6.97091003018116,1.8,7.));
#21888=CARTESIAN_POINT('Origin',(6.97091003018116,1.8,7.));
#21889=CARTESIAN_POINT('',(5.77091003018116,1.8,7.));
#26932=UNCERTAINTY_MEASURE_WITH_UNIT(LENGTH_MEASURE(0.001),#27070,
'DISTANCE_ACCURACY_VALUE',
'Maximum model space distance between geometric entities at asserted c
onnectivities');
#26992=UNCERTAINTY_MEASURE_WITH_UNIT(LENGTH_MEASURE(0.001),#27070,
'DISTANCE_ACCURACY_VALUE',
'Maximum model space distance between geometric entities at asserted c
onnectivities');
#27009=(
GEOMETRIC_REPRESENTATION_CONTEXT(3)
GLOBAL_UNCERTAINTY_ASSIGNED_CONTEXT((#26932))
GLOBAL_UNIT_ASSIGNED_CONTEXT((#27070,#27072,#27073))
REPRESENTATION_CONTEXT('','3D')
);
#27069=(
GEOMETRIC_REPRESENTATION_CONTEXT(3)
GLOBAL_UNCERTAINTY_ASSIGNED_CONTEXT((#26992))
GLOBAL_UNIT_ASSIGNED_CONTEXT((#27070,#27072,#27073))
REPRESENTATION_CONTEXT('','3D')
);
#27070=(
LENGTH_UNIT()
NAMED_UNIT(*)
SI_UNIT(.CENTI.,.METRE.)
);
#27072=(
NAMED_UNIT(*)
PLANE_ANGLE_UNIT()
SI_UNIT($,.RADIAN.)
);
#27073=(
NAMED_UNIT(*)
SI_UNIT($,.STERADIAN.)
SOLID_ANGLE_UNIT()
);
#27090=SHAPE_DEFINITION_REPRESENTATION(#27166,#27367);
#27166=PRODUCT_DEFINITION_SHAPE('',$,#27444);
#27367=SHAPE_REPRESENTATION('',(#14921),#27009);
#27427=PRODUCT_DEFINITION_CONTEXT('part definition',#27657,'design');
#27444=PRODUCT_DEFINITION('Output bearing cap (1)',
'Output bearing cap (1)',#27520,#27427);
#27520=PRODUCT_DEFINITION_FORMATION('',$,#27675);
#27657=APPLICATION_CONTEXT(
'Core Data for Automotive Mechanical Design Process');
#27658=PRODUCT_CONTEXT('part definition',#27657,'mechanical');
#27675=PRODUCT('Output bearing cap (1)','Output bearing cap (1)',
'Output bearing cap (1)',(#27658));
#27791=COLOUR_RGB('Grey',0.48,0.52,0.57);
#27792=FILL_AREA_STYLE_COLOUR('',#27791);
#27793=FILL_AREA_STYLE('',(#27792));
#27794=SURFACE_STYLE_FILL_AREA(#27793);
#27795=SURFACE_SIDE_STYLE('',(#27794));
#27796=SURFACE_STYLE_USAGE(.BOTH.,#27795);
#27797=PRESENTATION_STYLE_ASSIGNMENT((#27796));
ENDSEC;
END-ISO-10303-21;
